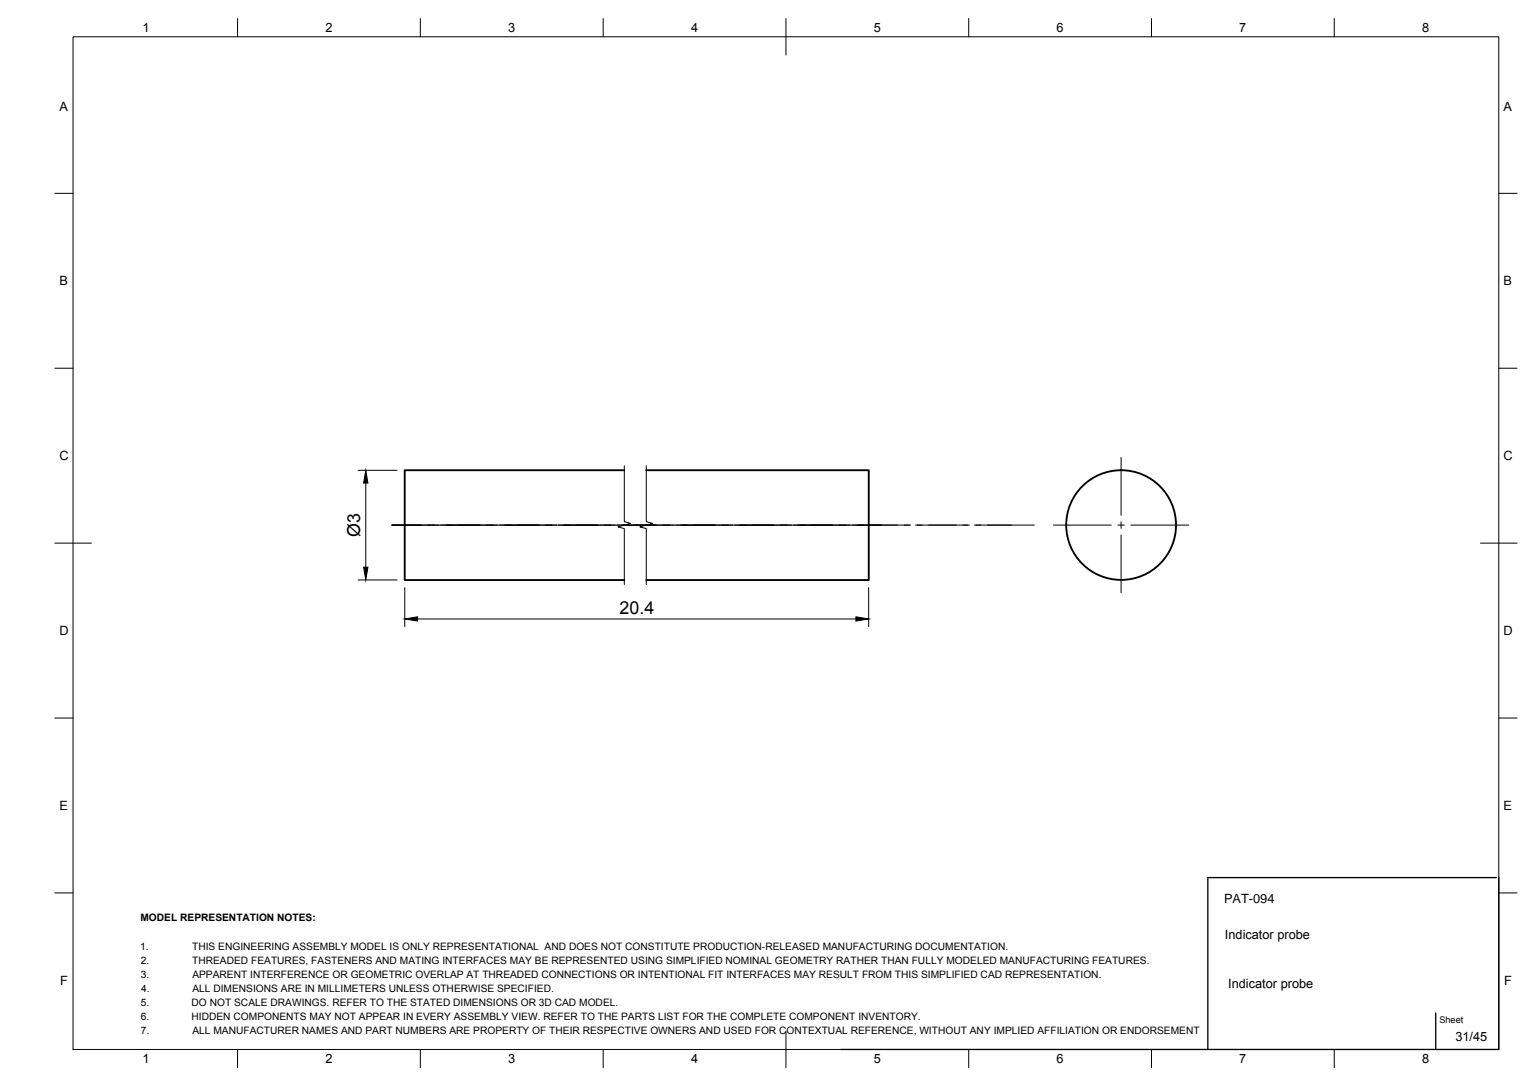
ISO-10303-21;
HEADER;
/* Generated by software containing ST-Developer
 * from STEP Tools, Inc. (www.steptools.com) 
 */

FILE_DESCRIPTION(
/* description */ ('Shaft runout checking stand'),
/* implementation_level */ '2;1');

FILE_NAME(
/* name */ 'Indicator probe.step',
/* time_stamp */ '2026-11-02T21:12:33-08:00',
/* author */ (''),
/* organization */ (''),
/* preprocessor_version */ 'ST-DEVELOPER v20.2',
/* originating_system */ 'Autodesk Translation Framework v15.17.0.0',
/* authorisation */ '');

FILE_SCHEMA (('AUTOMOTIVE_DESIGN { 1 0 10303 214 3 1 1 }'));
ENDSEC;

DATA;
#10=MECHANICAL_DESIGN_GEOMETRIC_PRESENTATION_REPRESENTATION('',(#493),#11748);
#407=SHAPE_REPRESENTATION_RELATIONSHIP('SRR','None',#11956,#450);
#450=ADVANCED_BREP_SHAPE_REPRESENTATION('',(#541),#11732);
#493=STYLED_ITEM('',(#12169),#541);
#541=MANIFOLD_SOLID_BREP('Body1',#6239);
#838=CIRCLE('',#7222,0.15);
#839=CIRCLE('',#7223,0.15);
#1012=CYLINDRICAL_SURFACE('',#7221,0.15);
#1325=FACE_OUTER_BOUND('',#1783,.T.);
#1326=FACE_OUTER_BOUND('',#1784,.T.);
#1327=FACE_OUTER_BOUND('',#1785,.T.);
#1783=EDGE_LOOP('',(#5308,#5309,#5310,#5311));
#1784=EDGE_LOOP('',(#5312));
#1785=EDGE_LOOP('',(#5313));
#2322=LINE('',#10890,#2789);
#2789=VECTOR('',#8907,0.15);
#3222=VERTEX_POINT('',#10887);
#3223=VERTEX_POINT('',#10889);
#3940=EDGE_CURVE('',#3222,#3222,#838,.T.);
#3941=EDGE_CURVE('',#3222,#3223,#2322,.T.);
#3942=EDGE_CURVE('',#3223,#3223,#839,.T.);
#5308=ORIENTED_EDGE('',*,*,#3940,.F.);
#5309=ORIENTED_EDGE('',*,*,#3941,.T.);
#5310=ORIENTED_EDGE('',*,*,#3942,.T.);
#5311=ORIENTED_EDGE('',*,*,#3941,.F.);
#5312=ORIENTED_EDGE('',*,*,#3940,.T.);
#5313=ORIENTED_EDGE('',*,*,#3942,.F.);
#5805=PLANE('',#7224);
#5806=PLANE('',#7225);
#6125=ADVANCED_FACE('',(#1325),#1012,.T.);
#6126=ADVANCED_FACE('',(#1326),#5805,.T.);
#6127=ADVANCED_FACE('',(#1327),#5806,.F.);
#6239=CLOSED_SHELL('',(#6125,#6126,#6127));
#7220=AXIS2_PLACEMENT_3D('',#10885,#8901,#8902);
#7221=AXIS2_PLACEMENT_3D('',#10886,#8903,#8904);
#7222=AXIS2_PLACEMENT_3D('',#10888,#8905,#8906);
#7223=AXIS2_PLACEMENT_3D('',#10891,#8908,#8909);
#7224=AXIS2_PLACEMENT_3D('',#10892,#8910,#8911);
#7225=AXIS2_PLACEMENT_3D('',#10893,#8912,#8913);
#8901=DIRECTION('axis',(0.,0.,1.));
#8902=DIRECTION('refdir',(1.,0.,0.));
#8903=DIRECTION('center_axis',(0.,0.,1.));
#8904=DIRECTION('ref_axis',(1.,0.,0.));
#8905=DIRECTION('center_axis',(0.,0.,1.));
#8906=DIRECTION('ref_axis',(1.,0.,0.));
#8907=DIRECTION('',(0.,0.,-1.));
#8908=DIRECTION('center_axis',(0.,0.,1.));
#8909=DIRECTION('ref_axis',(1.,0.,0.));
#8910=DIRECTION('center_axis',(0.,0.,1.));
#8911=DIRECTION('ref_axis',(1.,0.,0.));
#8912=DIRECTION('center_axis',(0.,0.,1.));
#8913=DIRECTION('ref_axis',(1.,0.,0.));
#10885=CARTESIAN_POINT('',(0.,0.,0.));
#10886=CARTESIAN_POINT('Origin',(0.,0.,7.95959179));
#10887=CARTESIAN_POINT('',(-0.15,-1.83697019872103E-17,10.));
#10888=CARTESIAN_POINT('Origin',(0.,0.,10.));
#10889=CARTESIAN_POINT('',(-0.15,-1.83697019872103E-17,7.95959179));
#10890=CARTESIAN_POINT('',(-0.15,-1.83697019872103E-17,7.95959179));
#10891=CARTESIAN_POINT('Origin',(0.,0.,7.95959179));
#10892=CARTESIAN_POINT('Origin',(0.,0.,10.));
#10893=CARTESIAN_POINT('Origin',(0.,0.,7.95959179));
#11683=UNCERTAINTY_MEASURE_WITH_UNIT(LENGTH_MEASURE(0.001),#11749,
'DISTANCE_ACCURACY_VALUE',
'Maximum model space distance between geometric entities at asserted c
onnectivities');
#11699=UNCERTAINTY_MEASURE_WITH_UNIT(LENGTH_MEASURE(0.001),#11749,
'DISTANCE_ACCURACY_VALUE',
'Maximum model space distance between geometric entities at asserted c
onnectivities');
#11732=(
GEOMETRIC_REPRESENTATION_CONTEXT(3)
GLOBAL_UNCERTAINTY_ASSIGNED_CONTEXT((#11683))
GLOBAL_UNIT_ASSIGNED_CONTEXT((#11749,#11751,#11752))
REPRESENTATION_CONTEXT('','3D')
);
#11748=(
GEOMETRIC_REPRESENTATION_CONTEXT(3)
GLOBAL_UNCERTAINTY_ASSIGNED_CONTEXT((#11699))
GLOBAL_UNIT_ASSIGNED_CONTEXT((#11749,#11751,#11752))
REPRESENTATION_CONTEXT('','3D')
);
#11749=(
LENGTH_UNIT()
NAMED_UNIT(*)
SI_UNIT(.CENTI.,.METRE.)
);
#11751=(
NAMED_UNIT(*)
PLANE_ANGLE_UNIT()
SI_UNIT($,.RADIAN.)
);
#11752=(
NAMED_UNIT(*)
SI_UNIT($,.STERADIAN.)
SOLID_ANGLE_UNIT()
);
#11785=SHAPE_DEFINITION_REPRESENTATION(#11833,#11956);
#11833=PRODUCT_DEFINITION_SHAPE('',$,#12005);
#11956=SHAPE_REPRESENTATION('',(#7220),#11732);
#11972=PRODUCT_DEFINITION_CONTEXT('part definition',#12118,'design');
#12005=PRODUCT_DEFINITION('Indicator probe','Indicator probe',#12053,#11972);
#12053=PRODUCT_DEFINITION_FORMATION('',$,#12152);
#12118=APPLICATION_CONTEXT(
'Core Data for Automotive Mechanical Design Process');
#12119=PRODUCT_CONTEXT('part definition',#12118,'mechanical');
#12152=PRODUCT('Indicator probe','Indicator probe','Indicator probe',(#12119));
#12169=PRESENTATION_STYLE_ASSIGNMENT((#12174));
#12174=SURFACE_STYLE_USAGE(.BOTH.,#12179);
#12179=SURFACE_SIDE_STYLE('',(#12184));
#12184=SURFACE_STYLE_FILL_AREA(#12189);
#12189=FILL_AREA_STYLE('CAD Library Painted - Engineering blue',(#12194));
#12194=FILL_AREA_STYLE_COLOUR('CAD Library Painted - Engineering blue',
#12199);
#12199=COLOUR_RGB('CAD Library Painted - Engineering blue',0.12156862745098,
0.356862745098039,0.6);
ENDSEC;
END-ISO-10303-21;
